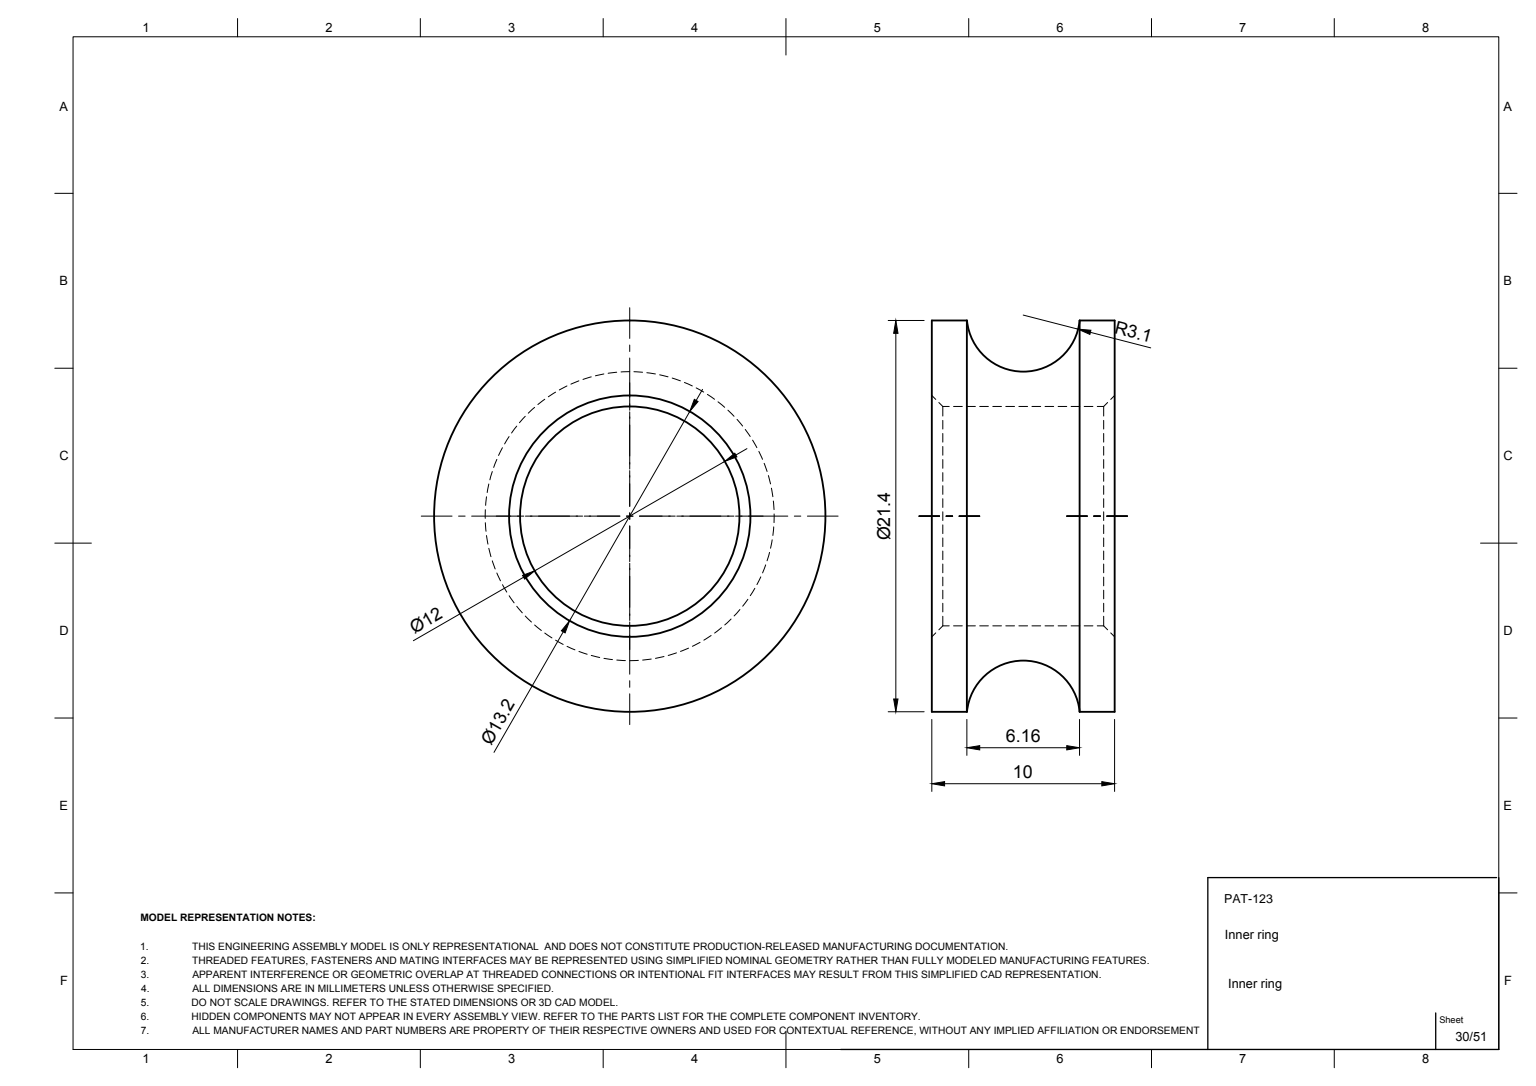
ISO-10303-21;
HEADER;
/* Generated by software containing ST-Developer
 * from STEP Tools, Inc. (www.steptools.com) 
 */

FILE_DESCRIPTION(
/* description */ ('Worm-less right-angle friction wheel drive'),
/* implementation_level */ '2;1');

FILE_NAME(
/* name */ 'Inner ring.step',
/* time_stamp */ '2026-10-28T03:22:36-07:00',
/* author */ (''),
/* organization */ (''),
/* preprocessor_version */ 'ST-DEVELOPER v20.2',
/* originating_system */ 'Autodesk Translation Framework v15.17.0.0',
/* authorisation */ '');

FILE_SCHEMA (('AUTOMOTIVE_DESIGN { 1 0 10303 214 3 1 1 }'));
ENDSEC;

DATA;
#10=MECHANICAL_DESIGN_GEOMETRIC_PRESENTATION_REPRESENTATION('',(#635),#17046);
#449=TOROIDAL_SURFACE('',#9263,1.1,0.309556);
#459=CONICAL_SURFACE('',#9274,0.63,0.785398163397448);
#460=CONICAL_SURFACE('',#9281,0.63,0.785398163397448);
#541=SHAPE_REPRESENTATION_RELATIONSHIP('SRR','None',#17285,#588);
#588=ADVANCED_BREP_SHAPE_REPRESENTATION('',(#688),#17021);
#635=STYLED_ITEM('',(#17591),#688);
#688=MANIFOLD_SOLID_BREP('Body1',#8191);
#906=FACE_BOUND('',#2121,.T.);
#907=FACE_BOUND('',#2124,.T.);
#1079=PLANE('',#9276);
#1080=PLANE('',#9279);
#1459=FACE_OUTER_BOUND('',#2116,.T.);
#1460=FACE_OUTER_BOUND('',#2117,.T.);
#1461=FACE_OUTER_BOUND('',#2118,.T.);
#1462=FACE_OUTER_BOUND('',#2119,.T.);
#1463=FACE_OUTER_BOUND('',#2120,.T.);
#1464=FACE_OUTER_BOUND('',#2122,.T.);
#1465=FACE_OUTER_BOUND('',#2123,.T.);
#1466=FACE_OUTER_BOUND('',#2125,.T.);
#2116=EDGE_LOOP('',(#6666,#6667,#6668,#6669,#6670,#6671));
#2117=EDGE_LOOP('',(#6672,#6673,#6674,#6675,#6676));
#2118=EDGE_LOOP('',(#6677,#6678,#6679,#6680));
#2119=EDGE_LOOP('',(#6681,#6682,#6683,#6684));
#2120=EDGE_LOOP('',(#6685));
#2121=EDGE_LOOP('',(#6686));
#2122=EDGE_LOOP('',(#6687,#6688,#6689,#6690,#6691));
#2123=EDGE_LOOP('',(#6692));
#2124=EDGE_LOOP('',(#6693));
#2125=EDGE_LOOP('',(#6694,#6695,#6696,#6697));
#2697=LINE('',#15408,#3237);
#2698=LINE('',#15414,#3238);
#2699=LINE('',#15418,#3239);
#2700=LINE('',#15424,#3240);
#2701=LINE('',#15429,#3241);
#3237=VECTOR('',#11149,1.070235);
#3238=VECTOR('',#11156,0.6);
#3239=VECTOR('',#11161,0.63);
#3240=VECTOR('',#11170,1.070235);
#3241=VECTOR('',#11177,0.63);
#3701=CIRCLE('',#9264,1.070235);
#3702=CIRCLE('',#9265,1.070235);
#3703=CIRCLE('',#9266,0.309556);
#3704=CIRCLE('',#9267,1.070235);
#3705=CIRCLE('',#9268,1.070235);
#3706=CIRCLE('',#9270,1.070235);
#3707=CIRCLE('',#9272,0.6);
#3708=CIRCLE('',#9273,0.6);
#3709=CIRCLE('',#9275,0.66);
#3710=CIRCLE('',#9278,1.070235);
#3711=CIRCLE('',#9280,0.66);
#4245=VERTEX_POINT('',#15397);
#4246=VERTEX_POINT('',#15398);
#4247=VERTEX_POINT('',#15401);
#4248=VERTEX_POINT('',#15403);
#4249=VERTEX_POINT('',#15407);
#4250=VERTEX_POINT('',#15411);
#4251=VERTEX_POINT('',#15413);
#4252=VERTEX_POINT('',#15417);
#4253=VERTEX_POINT('',#15422);
#4254=VERTEX_POINT('',#15426);
#5102=EDGE_CURVE('',#4245,#4246,#3701,.T.);
#5103=EDGE_CURVE('',#4246,#4245,#3702,.T.);
#5104=EDGE_CURVE('',#4246,#4247,#3703,.T.);
#5105=EDGE_CURVE('',#4248,#4247,#3704,.T.);
#5106=EDGE_CURVE('',#4247,#4248,#3705,.T.);
#5107=EDGE_CURVE('',#4248,#4249,#2697,.T.);
#5108=EDGE_CURVE('',#4249,#4249,#3706,.T.);
#5109=EDGE_CURVE('',#4250,#4250,#3707,.T.);
#5110=EDGE_CURVE('',#4250,#4251,#2698,.T.);
#5111=EDGE_CURVE('',#4251,#4251,#3708,.T.);
#5112=EDGE_CURVE('',#4251,#4252,#2699,.T.);
#5113=EDGE_CURVE('',#4252,#4252,#3709,.T.);
#5114=EDGE_CURVE('',#4253,#4253,#3710,.T.);
#5115=EDGE_CURVE('',#4253,#4245,#2700,.T.);
#5116=EDGE_CURVE('',#4254,#4254,#3711,.T.);
#5117=EDGE_CURVE('',#4254,#4250,#2701,.T.);
#6666=ORIENTED_EDGE('',*,*,#5102,.F.);
#6667=ORIENTED_EDGE('',*,*,#5103,.F.);
#6668=ORIENTED_EDGE('',*,*,#5104,.T.);
#6669=ORIENTED_EDGE('',*,*,#5105,.F.);
#6670=ORIENTED_EDGE('',*,*,#5106,.F.);
#6671=ORIENTED_EDGE('',*,*,#5104,.F.);
#6672=ORIENTED_EDGE('',*,*,#5105,.T.);
#6673=ORIENTED_EDGE('',*,*,#5106,.T.);
#6674=ORIENTED_EDGE('',*,*,#5107,.T.);
#6675=ORIENTED_EDGE('',*,*,#5108,.T.);
#6676=ORIENTED_EDGE('',*,*,#5107,.F.);
#6677=ORIENTED_EDGE('',*,*,#5109,.T.);
#6678=ORIENTED_EDGE('',*,*,#5110,.T.);
#6679=ORIENTED_EDGE('',*,*,#5111,.F.);
#6680=ORIENTED_EDGE('',*,*,#5110,.F.);
#6681=ORIENTED_EDGE('',*,*,#5111,.T.);
#6682=ORIENTED_EDGE('',*,*,#5112,.T.);
#6683=ORIENTED_EDGE('',*,*,#5113,.F.);
#6684=ORIENTED_EDGE('',*,*,#5112,.F.);
#6685=ORIENTED_EDGE('',*,*,#5108,.F.);
#6686=ORIENTED_EDGE('',*,*,#5113,.T.);
#6687=ORIENTED_EDGE('',*,*,#5114,.F.);
#6688=ORIENTED_EDGE('',*,*,#5115,.T.);
#6689=ORIENTED_EDGE('',*,*,#5102,.T.);
#6690=ORIENTED_EDGE('',*,*,#5103,.T.);
#6691=ORIENTED_EDGE('',*,*,#5115,.F.);
#6692=ORIENTED_EDGE('',*,*,#5114,.T.);
#6693=ORIENTED_EDGE('',*,*,#5116,.F.);
#6694=ORIENTED_EDGE('',*,*,#5116,.T.);
#6695=ORIENTED_EDGE('',*,*,#5117,.T.);
#6696=ORIENTED_EDGE('',*,*,#5109,.F.);
#6697=ORIENTED_EDGE('',*,*,#5117,.F.);
#7648=CYLINDRICAL_SURFACE('',#9269,1.070235);
#7649=CYLINDRICAL_SURFACE('',#9271,0.6);
#7650=CYLINDRICAL_SURFACE('',#9277,1.070235);
#7951=ADVANCED_FACE('',(#1459),#449,.F.);
#7952=ADVANCED_FACE('',(#1460),#7648,.T.);
#7953=ADVANCED_FACE('',(#1461),#7649,.F.);
#7954=ADVANCED_FACE('',(#1462),#459,.F.);
#7955=ADVANCED_FACE('',(#1463,#906),#1079,.T.);
#7956=ADVANCED_FACE('',(#1464),#7650,.T.);
#7957=ADVANCED_FACE('',(#1465,#907),#1080,.T.);
#7958=ADVANCED_FACE('',(#1466),#460,.F.);
#8191=CLOSED_SHELL('',(#7951,#7952,#7953,#7954,#7955,#7956,#7957,#7958));
#9262=AXIS2_PLACEMENT_3D('',#15395,#11133,#11134);
#9263=AXIS2_PLACEMENT_3D('',#15396,#11135,#11136);
#9264=AXIS2_PLACEMENT_3D('',#15399,#11137,#11138);
#9265=AXIS2_PLACEMENT_3D('',#15400,#11139,#11140);
#9266=AXIS2_PLACEMENT_3D('',#15402,#11141,#11142);
#9267=AXIS2_PLACEMENT_3D('',#15404,#11143,#11144);
#9268=AXIS2_PLACEMENT_3D('',#15405,#11145,#11146);
#9269=AXIS2_PLACEMENT_3D('',#15406,#11147,#11148);
#9270=AXIS2_PLACEMENT_3D('',#15409,#11150,#11151);
#9271=AXIS2_PLACEMENT_3D('',#15410,#11152,#11153);
#9272=AXIS2_PLACEMENT_3D('',#15412,#11154,#11155);
#9273=AXIS2_PLACEMENT_3D('',#15415,#11157,#11158);
#9274=AXIS2_PLACEMENT_3D('',#15416,#11159,#11160);
#9275=AXIS2_PLACEMENT_3D('',#15419,#11162,#11163);
#9276=AXIS2_PLACEMENT_3D('',#15420,#11164,#11165);
#9277=AXIS2_PLACEMENT_3D('',#15421,#11166,#11167);
#9278=AXIS2_PLACEMENT_3D('',#15423,#11168,#11169);
#9279=AXIS2_PLACEMENT_3D('',#15425,#11171,#11172);
#9280=AXIS2_PLACEMENT_3D('',#15427,#11173,#11174);
#9281=AXIS2_PLACEMENT_3D('',#15428,#11175,#11176);
#11133=DIRECTION('axis',(0.,0.,1.));
#11134=DIRECTION('refdir',(1.,0.,0.));
#11135=DIRECTION('center_axis',(0.,-1.,0.));
#11136=DIRECTION('ref_axis',(0.,0.,-1.));
#11137=DIRECTION('center_axis',(0.,-1.,0.));
#11138=DIRECTION('ref_axis',(1.,0.,0.));
#11139=DIRECTION('center_axis',(0.,-1.,0.));
#11140=DIRECTION('ref_axis',(1.,0.,0.));
#11141=DIRECTION('center_axis',(1.,0.,1.22464679914735E-16));
#11142=DIRECTION('ref_axis',(-1.22464679914735E-16,0.,1.));
#11143=DIRECTION('center_axis',(0.,1.,0.));
#11144=DIRECTION('ref_axis',(1.,0.,0.));
#11145=DIRECTION('center_axis',(0.,1.,0.));
#11146=DIRECTION('ref_axis',(1.,0.,0.));
#11147=DIRECTION('center_axis',(0.,-1.,0.));
#11148=DIRECTION('ref_axis',(1.,0.,0.));
#11149=DIRECTION('',(0.,1.,0.));
#11150=DIRECTION('center_axis',(0.,-1.,0.));
#11151=DIRECTION('ref_axis',(1.,0.,0.));
#11152=DIRECTION('center_axis',(0.,-1.,0.));
#11153=DIRECTION('ref_axis',(1.,0.,0.));
#11154=DIRECTION('center_axis',(0.,-1.,0.));
#11155=DIRECTION('ref_axis',(1.,0.,0.));
#11156=DIRECTION('',(0.,1.,0.));
#11157=DIRECTION('center_axis',(0.,-1.,0.));
#11158=DIRECTION('ref_axis',(1.,0.,0.));
#11159=DIRECTION('center_axis',(0.,1.,0.));
#11160=DIRECTION('ref_axis',(1.,0.,0.));
#11161=DIRECTION('',(-0.707106781186548,0.707106781186547,-8.65956056235493E-17));
#11162=DIRECTION('center_axis',(0.,-1.,0.));
#11163=DIRECTION('ref_axis',(1.,0.,0.));
#11164=DIRECTION('center_axis',(0.,1.,0.));
#11165=DIRECTION('ref_axis',(0.,0.,1.));
#11166=DIRECTION('center_axis',(0.,-1.,0.));
#11167=DIRECTION('ref_axis',(1.,0.,0.));
#11168=DIRECTION('center_axis',(0.,-1.,0.));
#11169=DIRECTION('ref_axis',(1.,0.,0.));
#11170=DIRECTION('',(0.,1.,0.));
#11171=DIRECTION('center_axis',(0.,-1.,0.));
#11172=DIRECTION('ref_axis',(0.,0.,-1.));
#11173=DIRECTION('center_axis',(0.,-1.,0.));
#11174=DIRECTION('ref_axis',(1.,0.,0.));
#11175=DIRECTION('center_axis',(0.,-1.,0.));
#11176=DIRECTION('ref_axis',(1.,0.,0.));
#11177=DIRECTION('',(0.707106781186548,0.707106781186547,8.65956056235493E-17));
#15395=CARTESIAN_POINT('',(0.,0.,0.));
#15396=CARTESIAN_POINT('Origin',(0.,0.,0.));
#15397=CARTESIAN_POINT('',(-1.070235,-0.308121667383195,-1.31065986708547E-16));
#15398=CARTESIAN_POINT('',(-1.31065986708547E-16,-0.308121667383195,1.070235));
#15399=CARTESIAN_POINT('Origin',(0.,-0.308121667383195,0.));
#15400=CARTESIAN_POINT('Origin',(0.,-0.308121667383195,0.));
#15401=CARTESIAN_POINT('',(-1.31065986708547E-16,0.308121667383195,1.070235));
#15402=CARTESIAN_POINT('Origin',(-1.34711147906209E-16,0.,1.1));
#15403=CARTESIAN_POINT('',(-1.070235,0.308121667383195,1.31065986708547E-16));
#15404=CARTESIAN_POINT('Origin',(0.,0.308121667383195,0.));
#15405=CARTESIAN_POINT('Origin',(0.,0.308121667383195,0.));
#15406=CARTESIAN_POINT('Origin',(0.,0.,0.));
#15407=CARTESIAN_POINT('',(-1.070235,0.5,-1.31065986708547E-16));
#15408=CARTESIAN_POINT('',(-1.070235,0.,-1.31065986708547E-16));
#15409=CARTESIAN_POINT('Origin',(0.,0.5,0.));
#15410=CARTESIAN_POINT('Origin',(0.,0.,0.));
#15411=CARTESIAN_POINT('',(-0.6,-0.44,-7.34788079488412E-17));
#15412=CARTESIAN_POINT('Origin',(0.,-0.44,0.));
#15413=CARTESIAN_POINT('',(-0.6,0.44,-7.34788079488412E-17));
#15414=CARTESIAN_POINT('',(-0.6,0.,-7.34788079488412E-17));
#15415=CARTESIAN_POINT('Origin',(0.,0.44,0.));
#15416=CARTESIAN_POINT('Origin',(0.,0.47,0.));
#15417=CARTESIAN_POINT('',(-0.66,0.5,-8.08266887437253E-17));
#15418=CARTESIAN_POINT('',(-0.63,0.47,-7.71527483462832E-17));
#15419=CARTESIAN_POINT('Origin',(0.,0.5,0.));
#15420=CARTESIAN_POINT('Origin',(1.070235,0.5,0.));
#15421=CARTESIAN_POINT('Origin',(0.,0.,0.));
#15422=CARTESIAN_POINT('',(-1.070235,-0.5,-1.31065986708547E-16));
#15423=CARTESIAN_POINT('Origin',(0.,-0.5,0.));
#15424=CARTESIAN_POINT('',(-1.070235,0.,-1.31065986708547E-16));
#15425=CARTESIAN_POINT('Origin',(0.66,-0.5,0.));
#15426=CARTESIAN_POINT('',(-0.66,-0.5,-8.08266887437253E-17));
#15427=CARTESIAN_POINT('Origin',(0.,-0.5,0.));
#15428=CARTESIAN_POINT('Origin',(0.,-0.47,0.));
#15429=CARTESIAN_POINT('',(-0.63,-0.47,-7.71527483462832E-17));
#16968=UNCERTAINTY_MEASURE_WITH_UNIT(LENGTH_MEASURE(0.001),#17047,
'DISTANCE_ACCURACY_VALUE',
'Maximum model space distance between geometric entities at asserted c
onnectivities');
#16993=UNCERTAINTY_MEASURE_WITH_UNIT(LENGTH_MEASURE(0.001),#17047,
'DISTANCE_ACCURACY_VALUE',
'Maximum model space distance between geometric entities at asserted c
onnectivities');
#17021=(
GEOMETRIC_REPRESENTATION_CONTEXT(3)
GLOBAL_UNCERTAINTY_ASSIGNED_CONTEXT((#16968))
GLOBAL_UNIT_ASSIGNED_CONTEXT((#17047,#17049,#17050))
REPRESENTATION_CONTEXT('','3D')
);
#17046=(
GEOMETRIC_REPRESENTATION_CONTEXT(3)
GLOBAL_UNCERTAINTY_ASSIGNED_CONTEXT((#16993))
GLOBAL_UNIT_ASSIGNED_CONTEXT((#17047,#17049,#17050))
REPRESENTATION_CONTEXT('','3D')
);
#17047=(
LENGTH_UNIT()
NAMED_UNIT(*)
SI_UNIT(.CENTI.,.METRE.)
);
#17049=(
NAMED_UNIT(*)
PLANE_ANGLE_UNIT()
SI_UNIT($,.RADIAN.)
);
#17050=(
NAMED_UNIT(*)
SI_UNIT($,.STERADIAN.)
SOLID_ANGLE_UNIT()
);
#17078=SHAPE_DEFINITION_REPRESENTATION(#17130,#17285);
#17130=PRODUCT_DEFINITION_SHAPE('',$,#17338);
#17285=SHAPE_REPRESENTATION('',(#9262),#17021);
#17310=PRODUCT_DEFINITION_CONTEXT('part definition',#17468,'design');
#17338=PRODUCT_DEFINITION('Inner ring','Inner ring',#17390,#17310);
#17390=PRODUCT_DEFINITION_FORMATION('',$,#17497);
#17468=APPLICATION_CONTEXT(
'Core Data for Automotive Mechanical Design Process');
#17469=PRODUCT_CONTEXT('part definition',#17468,'mechanical');
#17497=PRODUCT('Inner ring','Inner ring','Inner ring',(#17469));
#17585=COLOUR_RGB('Grey',0.48,0.52,0.57);
#17586=FILL_AREA_STYLE_COLOUR('',#17585);
#17587=FILL_AREA_STYLE('',(#17586));
#17588=SURFACE_STYLE_FILL_AREA(#17587);
#17589=SURFACE_SIDE_STYLE('',(#17588));
#17590=SURFACE_STYLE_USAGE(.BOTH.,#17589);
#17591=PRESENTATION_STYLE_ASSIGNMENT((#17590));
ENDSEC;
END-ISO-10303-21;
